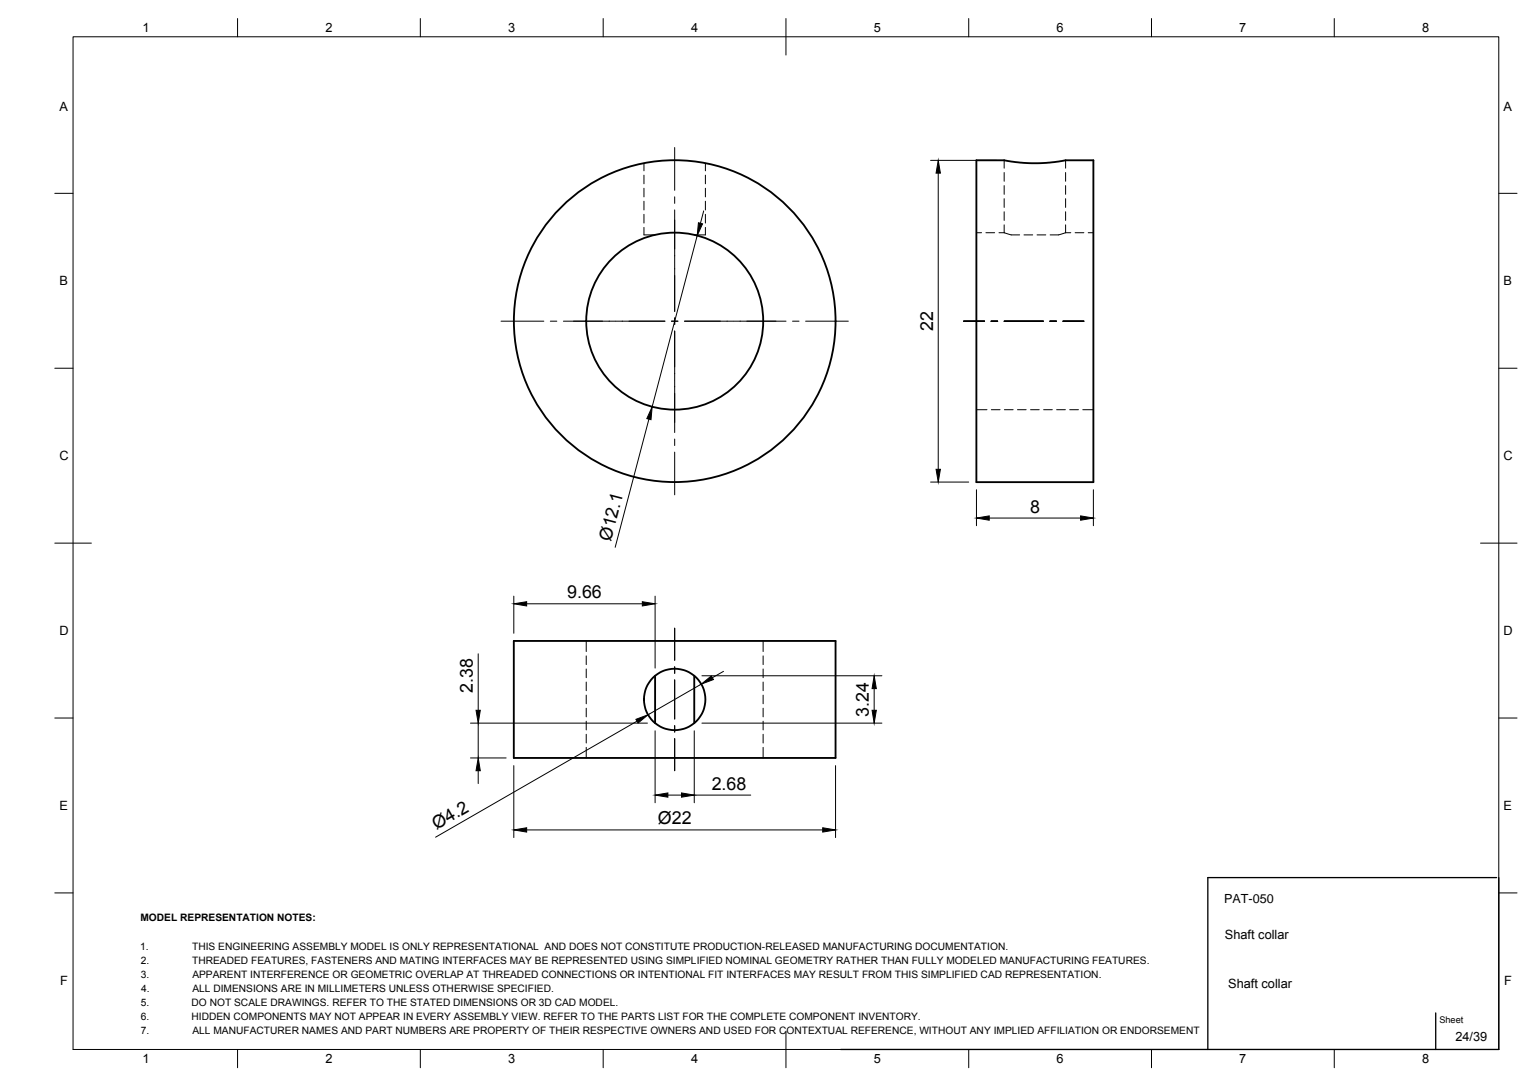
ISO-10303-21;
HEADER;
/* Generated by software containing ST-Developer
 * from STEP Tools, Inc. (www.steptools.com) 
 */

FILE_DESCRIPTION(
/* description */ ('Hand wheel with handle and shaft collar'),
/* implementation_level */ '2;1');

FILE_NAME(
/* name */ 'Shaft collar.step',
/* time_stamp */ '2026-10-28T03:23:19-07:00',
/* author */ (''),
/* organization */ (''),
/* preprocessor_version */ 'ST-DEVELOPER v20.2',
/* originating_system */ 'Autodesk Translation Framework v15.17.0.0',
/* authorisation */ '');

FILE_SCHEMA (('AUTOMOTIVE_DESIGN { 1 0 10303 214 3 1 1 }'));
ENDSEC;

DATA;
#10=MECHANICAL_DESIGN_GEOMETRIC_PRESENTATION_REPRESENTATION('',(#419),#10510);
#245=B_SPLINE_CURVE_WITH_KNOTS('',3,(#9365,#9366,#9367,#9368,#9369,#9370,
#9371,#9372,#9373,#9374),.UNSPECIFIED.,.F.,.F.,(4,2,2,2,4),(0.818088904349178,
0.878131747417165,0.957937926194036,1.03774410497091,1.09778694803889),
 .UNSPECIFIED.);
#246=B_SPLINE_CURVE_WITH_KNOTS('',3,(#9380,#9381,#9382,#9383,#9384,#9385,
#9386,#9387,#9388,#9389,#9390,#9391,#9392,#9393,#9394,#9395,#9396,#9397),
 .UNSPECIFIED.,.F.,.F.,(4,2,2,2,2,2,2,2,4),(0.,0.0793157643915218,0.158631528783044,
0.237943615933649,0.317255703084255,0.396567790234861,0.475879877385467,
0.555195641776989,0.634511406168511),.UNSPECIFIED.);
#247=B_SPLINE_CURVE_WITH_KNOTS('',3,(#9398,#9399,#9400,#9401,#9402,#9403,
#9404,#9405,#9406,#9407,#9408,#9409,#9410,#9411,#9412,#9413,#9414,#9415),
 .UNSPECIFIED.,.F.,.F.,(4,2,2,2,2,2,2,2,4),(0.634511406168511,0.713827170560032,
0.793142934951554,0.87245502210216,0.951767109252766,1.03107919640337,1.11039128355398,
1.1897070479455,1.26902281233702),.UNSPECIFIED.);
#248=B_SPLINE_CURVE_WITH_KNOTS('',3,(#9418,#9419,#9420,#9421,#9422,#9423,
#9424,#9425,#9426,#9427),.UNSPECIFIED.,.F.,.F.,(4,2,2,2,4),(0.17946362021982,
0.239506463287808,0.319312642064679,0.39911882084155,0.459161663909536),
 .UNSPECIFIED.);
#348=SHAPE_REPRESENTATION_RELATIONSHIP('SRR','None',#10666,#380);
#380=ADVANCED_BREP_SHAPE_REPRESENTATION('',(#465),#10493);
#419=STYLED_ITEM('',(#10908),#465);
#465=MANIFOLD_SOLID_BREP('Body1',#5319);
#566=FACE_BOUND('',#1339,.T.);
#567=FACE_BOUND('',#1341,.T.);
#568=FACE_BOUND('',#1343,.T.);
#569=FACE_BOUND('',#1345,.T.);
#689=PLANE('',#6072);
#690=PLANE('',#6077);
#691=PLANE('',#6084);
#692=PLANE('',#6085);
#936=FACE_OUTER_BOUND('',#1335,.T.);
#937=FACE_OUTER_BOUND('',#1336,.T.);
#938=FACE_OUTER_BOUND('',#1337,.T.);
#939=FACE_OUTER_BOUND('',#1338,.T.);
#940=FACE_OUTER_BOUND('',#1340,.T.);
#941=FACE_OUTER_BOUND('',#1342,.T.);
#942=FACE_OUTER_BOUND('',#1344,.T.);
#1335=EDGE_LOOP('',(#4315,#4316));
#1336=EDGE_LOOP('',(#4317,#4318,#4319,#4320,#4321,#4322,#4323,#4324,#4325));
#1337=EDGE_LOOP('',(#4326,#4327,#4328));
#1338=EDGE_LOOP('',(#4329,#4330,#4331,#4332));
#1339=EDGE_LOOP('',(#4333,#4334,#4335,#4336));
#1340=EDGE_LOOP('',(#4337,#4338,#4339,#4340));
#1341=EDGE_LOOP('',(#4341,#4342));
#1342=EDGE_LOOP('',(#4343));
#1343=EDGE_LOOP('',(#4344));
#1344=EDGE_LOOP('',(#4345));
#1345=EDGE_LOOP('',(#4346));
#1699=LINE('',#9361,#2009);
#1700=LINE('',#9378,#2010);
#1701=LINE('',#9429,#2011);
#1702=LINE('',#9434,#2012);
#1703=LINE('',#9440,#2013);
#2009=VECTOR('',#7357,1.);
#2010=VECTOR('',#7364,0.21);
#2011=VECTOR('',#7369,1.);
#2012=VECTOR('',#7374,0.605);
#2013=VECTOR('',#7381,1.1);
#2308=CIRCLE('',#6073,0.21);
#2309=CIRCLE('',#6075,0.21);
#2310=CIRCLE('',#6076,0.21);
#2311=CIRCLE('',#6079,0.605);
#2312=CIRCLE('',#6080,0.605);
#2313=CIRCLE('',#6082,1.1);
#2314=CIRCLE('',#6083,1.1);
#2704=VERTEX_POINT('',#9359);
#2705=VERTEX_POINT('',#9360);
#2706=VERTEX_POINT('',#9364);
#2707=VERTEX_POINT('',#9375);
#2708=VERTEX_POINT('',#9377);
#2709=VERTEX_POINT('',#9379);
#2710=VERTEX_POINT('',#9416);
#2711=VERTEX_POINT('',#9431);
#2712=VERTEX_POINT('',#9433);
#2713=VERTEX_POINT('',#9437);
#2714=VERTEX_POINT('',#9439);
#3275=EDGE_CURVE('',#2704,#2705,#1699,.T.);
#3276=EDGE_CURVE('',#2704,#2705,#2308,.T.);
#3277=EDGE_CURVE('',#2706,#2704,#245,.T.);
#3278=EDGE_CURVE('',#2707,#2706,#2309,.T.);
#3279=EDGE_CURVE('',#2707,#2708,#1700,.T.);
#3280=EDGE_CURVE('',#2709,#2708,#246,.T.);
#3281=EDGE_CURVE('',#2708,#2709,#247,.T.);
#3282=EDGE_CURVE('',#2710,#2707,#2310,.T.);
#3283=EDGE_CURVE('',#2705,#2710,#248,.T.);
#3284=EDGE_CURVE('',#2710,#2706,#1701,.T.);
#3285=EDGE_CURVE('',#2711,#2711,#2311,.T.);
#3286=EDGE_CURVE('',#2711,#2712,#1702,.T.);
#3287=EDGE_CURVE('',#2712,#2712,#2312,.T.);
#3288=EDGE_CURVE('',#2713,#2713,#2313,.T.);
#3289=EDGE_CURVE('',#2713,#2714,#1703,.T.);
#3290=EDGE_CURVE('',#2714,#2714,#2314,.T.);
#4315=ORIENTED_EDGE('',*,*,#3275,.F.);
#4316=ORIENTED_EDGE('',*,*,#3276,.T.);
#4317=ORIENTED_EDGE('',*,*,#3277,.F.);
#4318=ORIENTED_EDGE('',*,*,#3278,.F.);
#4319=ORIENTED_EDGE('',*,*,#3279,.T.);
#4320=ORIENTED_EDGE('',*,*,#3280,.F.);
#4321=ORIENTED_EDGE('',*,*,#3281,.F.);
#4322=ORIENTED_EDGE('',*,*,#3279,.F.);
#4323=ORIENTED_EDGE('',*,*,#3282,.F.);
#4324=ORIENTED_EDGE('',*,*,#3283,.F.);
#4325=ORIENTED_EDGE('',*,*,#3276,.F.);
#4326=ORIENTED_EDGE('',*,*,#3284,.F.);
#4327=ORIENTED_EDGE('',*,*,#3282,.T.);
#4328=ORIENTED_EDGE('',*,*,#3278,.T.);
#4329=ORIENTED_EDGE('',*,*,#3285,.F.);
#4330=ORIENTED_EDGE('',*,*,#3286,.T.);
#4331=ORIENTED_EDGE('',*,*,#3287,.T.);
#4332=ORIENTED_EDGE('',*,*,#3286,.F.);
#4333=ORIENTED_EDGE('',*,*,#3283,.T.);
#4334=ORIENTED_EDGE('',*,*,#3284,.T.);
#4335=ORIENTED_EDGE('',*,*,#3277,.T.);
#4336=ORIENTED_EDGE('',*,*,#3275,.T.);
#4337=ORIENTED_EDGE('',*,*,#3288,.F.);
#4338=ORIENTED_EDGE('',*,*,#3289,.T.);
#4339=ORIENTED_EDGE('',*,*,#3290,.T.);
#4340=ORIENTED_EDGE('',*,*,#3289,.F.);
#4341=ORIENTED_EDGE('',*,*,#3280,.T.);
#4342=ORIENTED_EDGE('',*,*,#3281,.T.);
#4343=ORIENTED_EDGE('',*,*,#3288,.T.);
#4344=ORIENTED_EDGE('',*,*,#3285,.T.);
#4345=ORIENTED_EDGE('',*,*,#3290,.F.);
#4346=ORIENTED_EDGE('',*,*,#3287,.F.);
#4938=CYLINDRICAL_SURFACE('',#6074,0.21);
#4939=CYLINDRICAL_SURFACE('',#6078,0.605);
#4940=CYLINDRICAL_SURFACE('',#6081,1.1);
#5148=ADVANCED_FACE('',(#936),#689,.T.);
#5149=ADVANCED_FACE('',(#937),#4938,.F.);
#5150=ADVANCED_FACE('',(#938),#690,.T.);
#5151=ADVANCED_FACE('',(#939,#566),#4939,.F.);
#5152=ADVANCED_FACE('',(#940,#567),#4940,.T.);
#5153=ADVANCED_FACE('',(#941,#568),#691,.T.);
#5154=ADVANCED_FACE('',(#942,#569),#692,.F.);
#5319=CLOSED_SHELL('',(#5148,#5149,#5150,#5151,#5152,#5153,#5154));
#6071=AXIS2_PLACEMENT_3D('',#9357,#7353,#7354);
#6072=AXIS2_PLACEMENT_3D('',#9358,#7355,#7356);
#6073=AXIS2_PLACEMENT_3D('',#9362,#7358,#7359);
#6074=AXIS2_PLACEMENT_3D('',#9363,#7360,#7361);
#6075=AXIS2_PLACEMENT_3D('',#9376,#7362,#7363);
#6076=AXIS2_PLACEMENT_3D('',#9417,#7365,#7366);
#6077=AXIS2_PLACEMENT_3D('',#9428,#7367,#7368);
#6078=AXIS2_PLACEMENT_3D('',#9430,#7370,#7371);
#6079=AXIS2_PLACEMENT_3D('',#9432,#7372,#7373);
#6080=AXIS2_PLACEMENT_3D('',#9435,#7375,#7376);
#6081=AXIS2_PLACEMENT_3D('',#9436,#7377,#7378);
#6082=AXIS2_PLACEMENT_3D('',#9438,#7379,#7380);
#6083=AXIS2_PLACEMENT_3D('',#9441,#7382,#7383);
#6084=AXIS2_PLACEMENT_3D('',#9442,#7384,#7385);
#6085=AXIS2_PLACEMENT_3D('',#9443,#7386,#7387);
#7353=DIRECTION('axis',(0.,0.,1.));
#7354=DIRECTION('refdir',(1.,0.,0.));
#7355=DIRECTION('center_axis',(0.,0.,1.));
#7356=DIRECTION('ref_axis',(1.,0.,0.));
#7357=DIRECTION('',(0.,1.,0.));
#7358=DIRECTION('center_axis',(0.,0.,1.));
#7359=DIRECTION('ref_axis',(1.,0.,0.));
#7360=DIRECTION('center_axis',(0.,0.,1.));
#7361=DIRECTION('ref_axis',(1.,0.,0.));
#7362=DIRECTION('center_axis',(0.,0.,1.));
#7363=DIRECTION('ref_axis',(1.,0.,0.));
#7364=DIRECTION('',(0.,0.,1.));
#7365=DIRECTION('center_axis',(0.,0.,1.));
#7366=DIRECTION('ref_axis',(1.,0.,0.));
#7367=DIRECTION('center_axis',(0.,0.,1.));
#7368=DIRECTION('ref_axis',(1.,0.,0.));
#7369=DIRECTION('',(0.,-1.,0.));
#7370=DIRECTION('center_axis',(0.,1.,0.));
#7371=DIRECTION('ref_axis',(1.,0.,0.));
#7372=DIRECTION('center_axis',(0.,-1.,0.));
#7373=DIRECTION('ref_axis',(1.,0.,0.));
#7374=DIRECTION('',(0.,-1.,0.));
#7375=DIRECTION('center_axis',(0.,-1.,0.));
#7376=DIRECTION('ref_axis',(1.,0.,0.));
#7377=DIRECTION('center_axis',(0.,1.,0.));
#7378=DIRECTION('ref_axis',(1.,0.,0.));
#7379=DIRECTION('center_axis',(0.,1.,0.));
#7380=DIRECTION('ref_axis',(1.,0.,0.));
#7381=DIRECTION('',(0.,-1.,0.));
#7382=DIRECTION('center_axis',(0.,1.,0.));
#7383=DIRECTION('ref_axis',(1.,0.,0.));
#7384=DIRECTION('center_axis',(0.,1.,0.));
#7385=DIRECTION('ref_axis',(1.,0.,0.));
#7386=DIRECTION('center_axis',(0.,1.,0.));
#7387=DIRECTION('ref_axis',(1.,0.,0.));
#9357=CARTESIAN_POINT('',(0.,0.,0.));
#9358=CARTESIAN_POINT('Origin',(0.,5.3,10.59));
#9359=CARTESIAN_POINT('',(0.133884278389952,5.13821310312636,10.59));
#9360=CARTESIAN_POINT('',(0.133884278389952,5.46178689687364,10.59));
#9361=CARTESIAN_POINT('',(0.133884278389952,4.9,10.59));
#9362=CARTESIAN_POINT('Origin',(0.,5.3,10.59));
#9363=CARTESIAN_POINT('Origin',(0.,5.3,10.59));
#9364=CARTESIAN_POINT('',(-0.133884278389952,5.13821310312636,10.59));
#9365=CARTESIAN_POINT('Ctrl Pts',(-0.133884278389952,5.13821310312636,10.59));
#9366=CARTESIAN_POINT('Ctrl Pts',(-0.118254395260799,5.12527883178237,10.5935467722442));
#9367=CARTESIAN_POINT('Ctrl Pts',(-0.100109787682297,5.11420068341256,10.5969822478996));
#9368=CARTESIAN_POINT('Ctrl Pts',(-0.0548298721325188,5.09536143894557,
10.6030741628997));
#9369=CARTESIAN_POINT('Ctrl Pts',(-0.0266020595922903,5.09,10.605));
#9370=CARTESIAN_POINT('Ctrl Pts',(0.0266020595922903,5.09,10.605));
#9371=CARTESIAN_POINT('Ctrl Pts',(0.0548298721325188,5.09536143894557,10.6030741628997));
#9372=CARTESIAN_POINT('Ctrl Pts',(0.100109787682297,5.11420068341256,10.5969822478996));
#9373=CARTESIAN_POINT('Ctrl Pts',(0.118254395260799,5.12527883178237,10.5935467722442));
#9374=CARTESIAN_POINT('Ctrl Pts',(0.133884278389952,5.13821310312636,10.59));
#9375=CARTESIAN_POINT('',(-0.21,5.3,10.59));
#9376=CARTESIAN_POINT('Origin',(0.,5.3,10.59));
#9377=CARTESIAN_POINT('',(-0.21,5.3,11.0797684937059));
#9378=CARTESIAN_POINT('',(-0.21,5.3,10.59));
#9379=CARTESIAN_POINT('',(0.21,5.3,11.0797684937059));
#9380=CARTESIAN_POINT('Ctrl Pts',(0.21,5.3,11.0797684937059));
#9381=CARTESIAN_POINT('Ctrl Pts',(0.21,5.27356141186949,11.0797684937059));
#9382=CARTESIAN_POINT('Ctrl Pts',(0.204702922670976,5.24540621874507,11.0808401566467));
#9383=CARTESIAN_POINT('Ctrl Pts',(0.183251796806354,5.19368655445866,11.0846831370713));
#9384=CARTESIAN_POINT('Ctrl Pts',(0.167101177357215,5.17011632925886,11.0873959305462));
#9385=CARTESIAN_POINT('Ctrl Pts',(0.129884533480965,5.13289968538261,11.0924663328912));
#9386=CARTESIAN_POINT('Ctrl Pts',(0.106313940757289,5.11674838983659,11.0951573889536));
#9387=CARTESIAN_POINT('Ctrl Pts',(0.0545930033295207,5.09529677343026,11.0989503922059));
#9388=CARTESIAN_POINT('Ctrl Pts',(0.0264373623835353,5.09,11.1));
#9389=CARTESIAN_POINT('Ctrl Pts',(-0.0264373623835352,5.09,11.1));
#9390=CARTESIAN_POINT('Ctrl Pts',(-0.0545930033295207,5.09529677343026,
11.0989503922059));
#9391=CARTESIAN_POINT('Ctrl Pts',(-0.106313940757289,5.11674838983659,11.0951573889536));
#9392=CARTESIAN_POINT('Ctrl Pts',(-0.129884533480965,5.13289968538261,11.0924663328912));
#9393=CARTESIAN_POINT('Ctrl Pts',(-0.167101177357215,5.17011632925886,11.0873959305462));
#9394=CARTESIAN_POINT('Ctrl Pts',(-0.183251796806354,5.19368655445866,11.0846831370713));
#9395=CARTESIAN_POINT('Ctrl Pts',(-0.204702922670976,5.24540621874507,11.0808401566467));
#9396=CARTESIAN_POINT('Ctrl Pts',(-0.21,5.27356141186949,11.0797684937059));
#9397=CARTESIAN_POINT('Ctrl Pts',(-0.21,5.3,11.0797684937059));
#9398=CARTESIAN_POINT('Ctrl Pts',(-0.21,5.3,11.0797684937059));
#9399=CARTESIAN_POINT('Ctrl Pts',(-0.21,5.32643858813051,11.0797684937059));
#9400=CARTESIAN_POINT('Ctrl Pts',(-0.204702922670976,5.35459378125493,11.0808401566467));
#9401=CARTESIAN_POINT('Ctrl Pts',(-0.183251796806354,5.40631344554134,11.0846831370713));
#9402=CARTESIAN_POINT('Ctrl Pts',(-0.167101177357215,5.42988367074114,11.0873959305462));
#9403=CARTESIAN_POINT('Ctrl Pts',(-0.129884533480965,5.46710031461738,11.0924663328912));
#9404=CARTESIAN_POINT('Ctrl Pts',(-0.106313940757289,5.48325161016341,11.0951573889536));
#9405=CARTESIAN_POINT('Ctrl Pts',(-0.0545930033295208,5.50470322656974,
11.0989503922059));
#9406=CARTESIAN_POINT('Ctrl Pts',(-0.0264373623835353,5.51,11.1));
#9407=CARTESIAN_POINT('Ctrl Pts',(0.0264373623835352,5.51,11.1));
#9408=CARTESIAN_POINT('Ctrl Pts',(0.0545930033295208,5.50470322656974,11.0989503922059));
#9409=CARTESIAN_POINT('Ctrl Pts',(0.106313940757289,5.48325161016341,11.0951573889536));
#9410=CARTESIAN_POINT('Ctrl Pts',(0.129884533480965,5.46710031461738,11.0924663328912));
#9411=CARTESIAN_POINT('Ctrl Pts',(0.167101177357214,5.42988367074114,11.0873959305462));
#9412=CARTESIAN_POINT('Ctrl Pts',(0.183251796806354,5.40631344554134,11.0846831370713));
#9413=CARTESIAN_POINT('Ctrl Pts',(0.204702922670976,5.35459378125493,11.0808401566467));
#9414=CARTESIAN_POINT('Ctrl Pts',(0.21,5.32643858813051,11.0797684937059));
#9415=CARTESIAN_POINT('Ctrl Pts',(0.21,5.3,11.0797684937059));
#9416=CARTESIAN_POINT('',(-0.133884278389952,5.46178689687364,10.59));
#9417=CARTESIAN_POINT('Origin',(0.,5.3,10.59));
#9418=CARTESIAN_POINT('Ctrl Pts',(0.133884278389952,5.46178689687364,10.59));
#9419=CARTESIAN_POINT('Ctrl Pts',(0.118254395260798,5.47472116821763,10.5935467722442));
#9420=CARTESIAN_POINT('Ctrl Pts',(0.100109787682297,5.48579931658744,10.5969822478996));
#9421=CARTESIAN_POINT('Ctrl Pts',(0.0548298721325188,5.50463856105443,10.6030741628997));
#9422=CARTESIAN_POINT('Ctrl Pts',(0.0266020595922903,5.51,10.605));
#9423=CARTESIAN_POINT('Ctrl Pts',(-0.0266020595922903,5.51,10.605));
#9424=CARTESIAN_POINT('Ctrl Pts',(-0.0548298721325188,5.50463856105443,
10.6030741628997));
#9425=CARTESIAN_POINT('Ctrl Pts',(-0.100109787682297,5.48579931658744,10.5969822478996));
#9426=CARTESIAN_POINT('Ctrl Pts',(-0.118254395260799,5.47472116821763,10.5935467722442));
#9427=CARTESIAN_POINT('Ctrl Pts',(-0.133884278389952,5.46178689687364,10.59));
#9428=CARTESIAN_POINT('Origin',(0.,5.3,10.59));
#9429=CARTESIAN_POINT('',(-0.133884278389952,4.9,10.59));
#9430=CARTESIAN_POINT('Origin',(0.,4.9,10.));
#9431=CARTESIAN_POINT('',(-0.605,5.7,10.));
#9432=CARTESIAN_POINT('Origin',(0.,5.7,10.));
#9433=CARTESIAN_POINT('',(-0.605,4.9,10.));
#9434=CARTESIAN_POINT('',(-0.605,4.9,10.));
#9435=CARTESIAN_POINT('Origin',(0.,4.9,10.));
#9436=CARTESIAN_POINT('Origin',(0.,4.9,10.));
#9437=CARTESIAN_POINT('',(-1.1,5.7,10.));
#9438=CARTESIAN_POINT('Origin',(0.,5.7,10.));
#9439=CARTESIAN_POINT('',(-1.1,4.9,10.));
#9440=CARTESIAN_POINT('',(-1.1,4.9,10.));
#9441=CARTESIAN_POINT('Origin',(0.,4.9,10.));
#9442=CARTESIAN_POINT('Origin',(0.,5.7,10.));
#9443=CARTESIAN_POINT('Origin',(0.,4.9,10.));
#10454=UNCERTAINTY_MEASURE_WITH_UNIT(LENGTH_MEASURE(0.001),#10511,
'DISTANCE_ACCURACY_VALUE',
'Maximum model space distance between geometric entities at asserted c
onnectivities');
#10471=UNCERTAINTY_MEASURE_WITH_UNIT(LENGTH_MEASURE(0.001),#10511,
'DISTANCE_ACCURACY_VALUE',
'Maximum model space distance between geometric entities at asserted c
onnectivities');
#10493=(
GEOMETRIC_REPRESENTATION_CONTEXT(3)
GLOBAL_UNCERTAINTY_ASSIGNED_CONTEXT((#10454))
GLOBAL_UNIT_ASSIGNED_CONTEXT((#10511,#10513,#10514))
REPRESENTATION_CONTEXT('','3D')
);
#10510=(
GEOMETRIC_REPRESENTATION_CONTEXT(3)
GLOBAL_UNCERTAINTY_ASSIGNED_CONTEXT((#10471))
GLOBAL_UNIT_ASSIGNED_CONTEXT((#10511,#10513,#10514))
REPRESENTATION_CONTEXT('','3D')
);
#10511=(
LENGTH_UNIT()
NAMED_UNIT(*)
SI_UNIT(.CENTI.,.METRE.)
);
#10513=(
NAMED_UNIT(*)
PLANE_ANGLE_UNIT()
SI_UNIT($,.RADIAN.)
);
#10514=(
NAMED_UNIT(*)
SI_UNIT($,.STERADIAN.)
SOLID_ANGLE_UNIT()
);
#10536=SHAPE_DEFINITION_REPRESENTATION(#10579,#10666);
#10579=PRODUCT_DEFINITION_SHAPE('',$,#10705);
#10666=SHAPE_REPRESENTATION('',(#6071),#10493);
#10683=PRODUCT_DEFINITION_CONTEXT('part definition',#10799,'design');
#10705=PRODUCT_DEFINITION('Shaft collar','Shaft collar',#10743,#10683);
#10743=PRODUCT_DEFINITION_FORMATION('',$,#10822);
#10799=APPLICATION_CONTEXT(
'Core Data for Automotive Mechanical Design Process');
#10800=PRODUCT_CONTEXT('part definition',#10799,'mechanical');
#10822=PRODUCT('Shaft collar','Shaft collar','Shaft collar',(#10800));
#10902=COLOUR_RGB('Grey',0.48,0.52,0.57);
#10903=FILL_AREA_STYLE_COLOUR('',#10902);
#10904=FILL_AREA_STYLE('',(#10903));
#10905=SURFACE_STYLE_FILL_AREA(#10904);
#10906=SURFACE_SIDE_STYLE('',(#10905));
#10907=SURFACE_STYLE_USAGE(.BOTH.,#10906);
#10908=PRESENTATION_STYLE_ASSIGNMENT((#10907));
ENDSEC;
END-ISO-10303-21;
